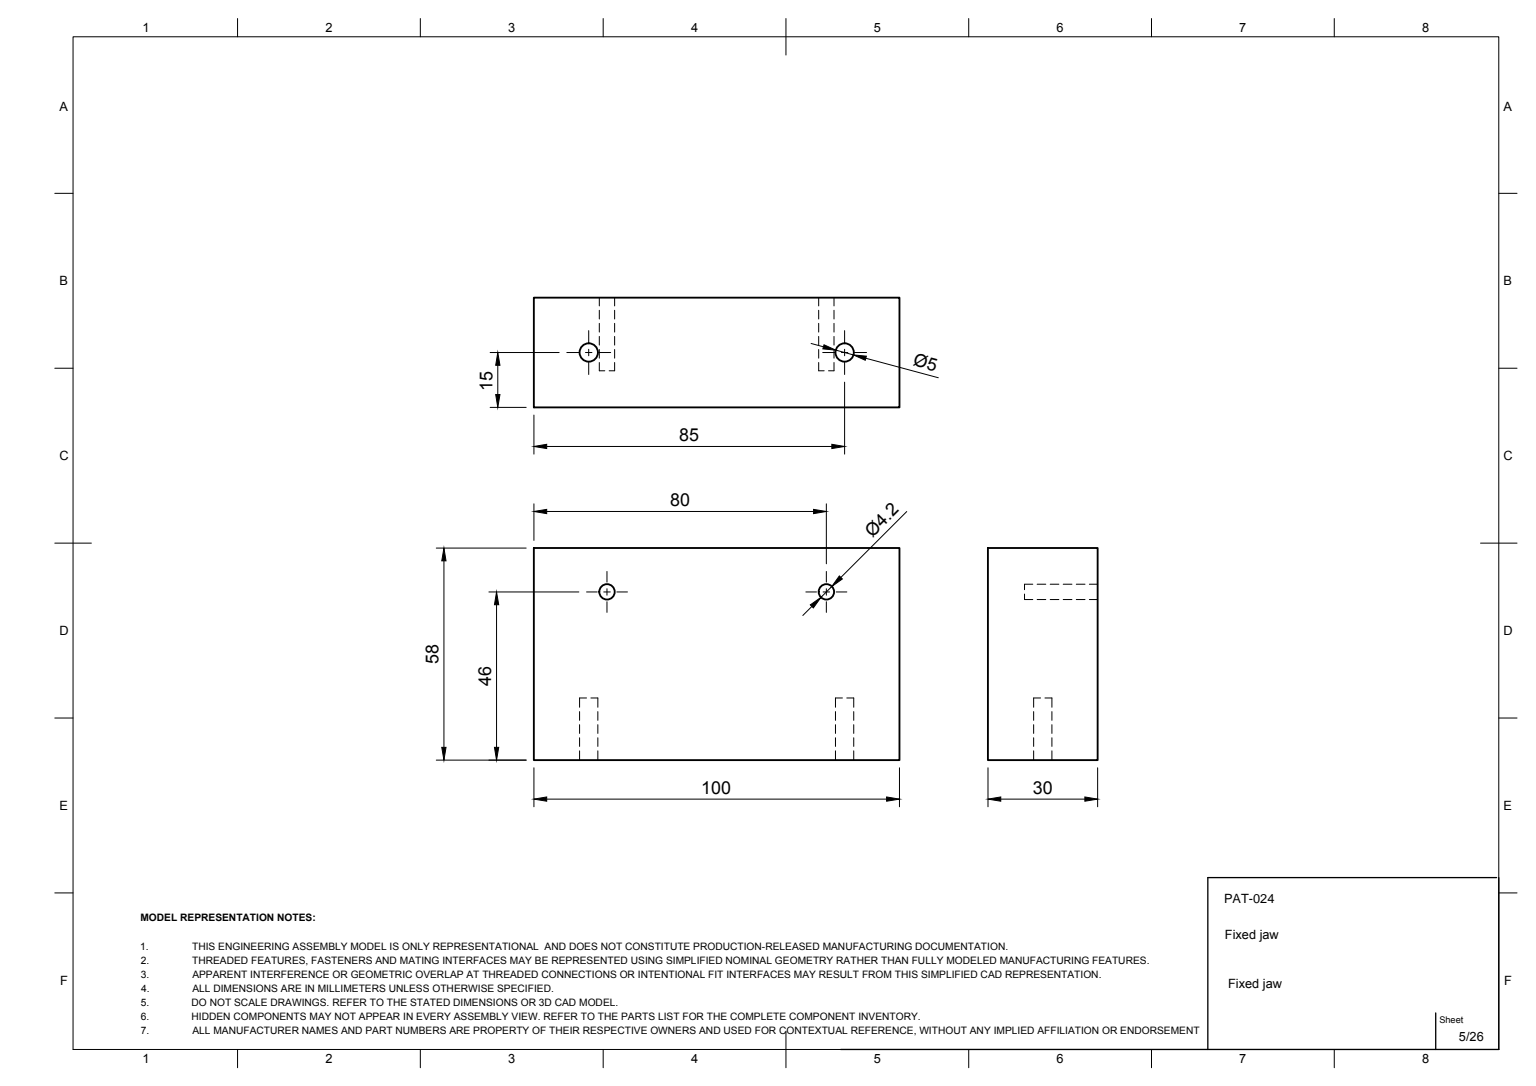
ISO-10303-21;
HEADER;
/* Generated by software containing ST-Developer
 * from STEP Tools, Inc. (www.steptools.com) 
 */

FILE_DESCRIPTION(
/* description */ ('Compact handwheel screw vise'),
/* implementation_level */ '2;1');

FILE_NAME(
/* name */ 'Fixed jaw.step',
/* time_stamp */ '2026-10-29T16:08:22-07:00',
/* author */ (''),
/* organization */ (''),
/* preprocessor_version */ 'ST-DEVELOPER v20.2',
/* originating_system */ 'Autodesk Translation Framework v15.17.0.0',
/* authorisation */ '');

FILE_SCHEMA (('AUTOMOTIVE_DESIGN { 1 0 10303 214 3 1 1 }'));
ENDSEC;

DATA;
#10=MECHANICAL_DESIGN_GEOMETRIC_PRESENTATION_REPRESENTATION('',(#646),#25074);
#590=SHAPE_REPRESENTATION_RELATIONSHIP('SRR','None',#25198,#618);
#618=ADVANCED_BREP_SHAPE_REPRESENTATION('',(#682),#25045);
#646=STYLED_ITEM('',(#25425),#682);
#682=MANIFOLD_SOLID_BREP('Body1',#8054);
#729=FACE_BOUND('',#1534,.T.);
#730=FACE_BOUND('',#1535,.T.);
#731=FACE_BOUND('',#1540,.T.);
#732=FACE_BOUND('',#1541,.T.);
#837=PLANE('',#8454);
#838=PLANE('',#8458);
#839=PLANE('',#8462);
#840=PLANE('',#8466);
#841=PLANE('',#8467);
#842=PLANE('',#8468);
#843=PLANE('',#8469);
#844=PLANE('',#8470);
#845=PLANE('',#8471);
#846=PLANE('',#8472);
#1037=FACE_OUTER_BOUND('',#1524,.T.);
#1038=FACE_OUTER_BOUND('',#1525,.T.);
#1039=FACE_OUTER_BOUND('',#1526,.T.);
#1040=FACE_OUTER_BOUND('',#1527,.T.);
#1041=FACE_OUTER_BOUND('',#1528,.T.);
#1042=FACE_OUTER_BOUND('',#1529,.T.);
#1043=FACE_OUTER_BOUND('',#1530,.T.);
#1044=FACE_OUTER_BOUND('',#1531,.T.);
#1045=FACE_OUTER_BOUND('',#1532,.T.);
#1046=FACE_OUTER_BOUND('',#1533,.T.);
#1047=FACE_OUTER_BOUND('',#1536,.T.);
#1048=FACE_OUTER_BOUND('',#1537,.T.);
#1049=FACE_OUTER_BOUND('',#1538,.T.);
#1050=FACE_OUTER_BOUND('',#1539,.T.);
#1524=EDGE_LOOP('',(#5267,#5268,#5269,#5270));
#1525=EDGE_LOOP('',(#5271));
#1526=EDGE_LOOP('',(#5272,#5273,#5274,#5275));
#1527=EDGE_LOOP('',(#5276));
#1528=EDGE_LOOP('',(#5277,#5278,#5279,#5280));
#1529=EDGE_LOOP('',(#5281));
#1530=EDGE_LOOP('',(#5282,#5283,#5284,#5285));
#1531=EDGE_LOOP('',(#5286));
#1532=EDGE_LOOP('',(#5287,#5288,#5289,#5290));
#1533=EDGE_LOOP('',(#5291,#5292,#5293,#5294));
#1534=EDGE_LOOP('',(#5295));
#1535=EDGE_LOOP('',(#5296));
#1536=EDGE_LOOP('',(#5297,#5298,#5299,#5300));
#1537=EDGE_LOOP('',(#5301,#5302,#5303,#5304));
#1538=EDGE_LOOP('',(#5305,#5306,#5307,#5308));
#1539=EDGE_LOOP('',(#5309,#5310,#5311,#5312));
#1540=EDGE_LOOP('',(#5313));
#1541=EDGE_LOOP('',(#5314));
#2096=LINE('',#11442,#2604);
#2097=LINE('',#11449,#2605);
#2098=LINE('',#11456,#2606);
#2099=LINE('',#11463,#2607);
#2100=LINE('',#11469,#2608);
#2101=LINE('',#11471,#2609);
#2102=LINE('',#11473,#2610);
#2103=LINE('',#11474,#2611);
#2104=LINE('',#11477,#2612);
#2105=LINE('',#11479,#2613);
#2106=LINE('',#11480,#2614);
#2107=LINE('',#11483,#2615);
#2108=LINE('',#11485,#2616);
#2109=LINE('',#11486,#2617);
#2110=LINE('',#11488,#2618);
#2111=LINE('',#11489,#2619);
#2604=VECTOR('',#9342,0.21);
#2605=VECTOR('',#9351,0.21);
#2606=VECTOR('',#9360,0.25);
#2607=VECTOR('',#9369,0.25);
#2608=VECTOR('',#9376,1.);
#2609=VECTOR('',#9377,1.);
#2610=VECTOR('',#9378,1.);
#2611=VECTOR('',#9379,1.);
#2612=VECTOR('',#9382,1.);
#2613=VECTOR('',#9383,1.);
#2614=VECTOR('',#9384,1.);
#2615=VECTOR('',#9387,1.);
#2616=VECTOR('',#9388,1.);
#2617=VECTOR('',#9389,1.);
#2618=VECTOR('',#9392,1.);
#2619=VECTOR('',#9393,1.);
#3098=CIRCLE('',#8452,0.21);
#3099=CIRCLE('',#8453,0.21);
#3100=CIRCLE('',#8456,0.21);
#3101=CIRCLE('',#8457,0.21);
#3102=CIRCLE('',#8460,0.25);
#3103=CIRCLE('',#8461,0.25);
#3104=CIRCLE('',#8464,0.25);
#3105=CIRCLE('',#8465,0.25);
#3369=VERTEX_POINT('',#11439);
#3370=VERTEX_POINT('',#11441);
#3371=VERTEX_POINT('',#11446);
#3372=VERTEX_POINT('',#11448);
#3373=VERTEX_POINT('',#11453);
#3374=VERTEX_POINT('',#11455);
#3375=VERTEX_POINT('',#11460);
#3376=VERTEX_POINT('',#11462);
#3377=VERTEX_POINT('',#11467);
#3378=VERTEX_POINT('',#11468);
#3379=VERTEX_POINT('',#11470);
#3380=VERTEX_POINT('',#11472);
#3381=VERTEX_POINT('',#11476);
#3382=VERTEX_POINT('',#11478);
#3383=VERTEX_POINT('',#11482);
#3384=VERTEX_POINT('',#11484);
#4120=EDGE_CURVE('',#3369,#3369,#3098,.T.);
#4121=EDGE_CURVE('',#3369,#3370,#2096,.T.);
#4122=EDGE_CURVE('',#3370,#3370,#3099,.T.);
#4123=EDGE_CURVE('',#3371,#3371,#3100,.T.);
#4124=EDGE_CURVE('',#3371,#3372,#2097,.T.);
#4125=EDGE_CURVE('',#3372,#3372,#3101,.T.);
#4126=EDGE_CURVE('',#3373,#3373,#3102,.T.);
#4127=EDGE_CURVE('',#3373,#3374,#2098,.T.);
#4128=EDGE_CURVE('',#3374,#3374,#3103,.T.);
#4129=EDGE_CURVE('',#3375,#3375,#3104,.T.);
#4130=EDGE_CURVE('',#3375,#3376,#2099,.T.);
#4131=EDGE_CURVE('',#3376,#3376,#3105,.T.);
#4132=EDGE_CURVE('',#3377,#3378,#2100,.T.);
#4133=EDGE_CURVE('',#3378,#3379,#2101,.T.);
#4134=EDGE_CURVE('',#3380,#3379,#2102,.T.);
#4135=EDGE_CURVE('',#3377,#3380,#2103,.T.);
#4136=EDGE_CURVE('',#3381,#3377,#2104,.T.);
#4137=EDGE_CURVE('',#3382,#3380,#2105,.T.);
#4138=EDGE_CURVE('',#3381,#3382,#2106,.T.);
#4139=EDGE_CURVE('',#3383,#3381,#2107,.T.);
#4140=EDGE_CURVE('',#3384,#3382,#2108,.T.);
#4141=EDGE_CURVE('',#3383,#3384,#2109,.T.);
#4142=EDGE_CURVE('',#3378,#3383,#2110,.T.);
#4143=EDGE_CURVE('',#3379,#3384,#2111,.T.);
#5267=ORIENTED_EDGE('',*,*,#4120,.F.);
#5268=ORIENTED_EDGE('',*,*,#4121,.T.);
#5269=ORIENTED_EDGE('',*,*,#4122,.F.);
#5270=ORIENTED_EDGE('',*,*,#4121,.F.);
#5271=ORIENTED_EDGE('',*,*,#4120,.T.);
#5272=ORIENTED_EDGE('',*,*,#4123,.F.);
#5273=ORIENTED_EDGE('',*,*,#4124,.T.);
#5274=ORIENTED_EDGE('',*,*,#4125,.F.);
#5275=ORIENTED_EDGE('',*,*,#4124,.F.);
#5276=ORIENTED_EDGE('',*,*,#4123,.T.);
#5277=ORIENTED_EDGE('',*,*,#4126,.F.);
#5278=ORIENTED_EDGE('',*,*,#4127,.T.);
#5279=ORIENTED_EDGE('',*,*,#4128,.T.);
#5280=ORIENTED_EDGE('',*,*,#4127,.F.);
#5281=ORIENTED_EDGE('',*,*,#4128,.F.);
#5282=ORIENTED_EDGE('',*,*,#4129,.F.);
#5283=ORIENTED_EDGE('',*,*,#4130,.T.);
#5284=ORIENTED_EDGE('',*,*,#4131,.T.);
#5285=ORIENTED_EDGE('',*,*,#4130,.F.);
#5286=ORIENTED_EDGE('',*,*,#4131,.F.);
#5287=ORIENTED_EDGE('',*,*,#4132,.T.);
#5288=ORIENTED_EDGE('',*,*,#4133,.T.);
#5289=ORIENTED_EDGE('',*,*,#4134,.F.);
#5290=ORIENTED_EDGE('',*,*,#4135,.F.);
#5291=ORIENTED_EDGE('',*,*,#4136,.T.);
#5292=ORIENTED_EDGE('',*,*,#4135,.T.);
#5293=ORIENTED_EDGE('',*,*,#4137,.F.);
#5294=ORIENTED_EDGE('',*,*,#4138,.F.);
#5295=ORIENTED_EDGE('',*,*,#4122,.T.);
#5296=ORIENTED_EDGE('',*,*,#4125,.T.);
#5297=ORIENTED_EDGE('',*,*,#4139,.T.);
#5298=ORIENTED_EDGE('',*,*,#4138,.T.);
#5299=ORIENTED_EDGE('',*,*,#4140,.F.);
#5300=ORIENTED_EDGE('',*,*,#4141,.F.);
#5301=ORIENTED_EDGE('',*,*,#4142,.T.);
#5302=ORIENTED_EDGE('',*,*,#4141,.T.);
#5303=ORIENTED_EDGE('',*,*,#4143,.F.);
#5304=ORIENTED_EDGE('',*,*,#4133,.F.);
#5305=ORIENTED_EDGE('',*,*,#4143,.T.);
#5306=ORIENTED_EDGE('',*,*,#4140,.T.);
#5307=ORIENTED_EDGE('',*,*,#4137,.T.);
#5308=ORIENTED_EDGE('',*,*,#4134,.T.);
#5309=ORIENTED_EDGE('',*,*,#4142,.F.);
#5310=ORIENTED_EDGE('',*,*,#4132,.F.);
#5311=ORIENTED_EDGE('',*,*,#4136,.F.);
#5312=ORIENTED_EDGE('',*,*,#4139,.F.);
#5313=ORIENTED_EDGE('',*,*,#4126,.T.);
#5314=ORIENTED_EDGE('',*,*,#4129,.T.);
#7355=CYLINDRICAL_SURFACE('',#8451,0.21);
#7356=CYLINDRICAL_SURFACE('',#8455,0.21);
#7357=CYLINDRICAL_SURFACE('',#8459,0.25);
#7358=CYLINDRICAL_SURFACE('',#8463,0.25);
#7607=ADVANCED_FACE('',(#1037),#7355,.F.);
#7608=ADVANCED_FACE('',(#1038),#837,.T.);
#7609=ADVANCED_FACE('',(#1039),#7356,.F.);
#7610=ADVANCED_FACE('',(#1040),#838,.T.);
#7611=ADVANCED_FACE('',(#1041),#7357,.F.);
#7612=ADVANCED_FACE('',(#1042),#839,.F.);
#7613=ADVANCED_FACE('',(#1043),#7358,.F.);
#7614=ADVANCED_FACE('',(#1044),#840,.F.);
#7615=ADVANCED_FACE('',(#1045),#841,.T.);
#7616=ADVANCED_FACE('',(#1046,#729,#730),#842,.T.);
#7617=ADVANCED_FACE('',(#1047),#843,.T.);
#7618=ADVANCED_FACE('',(#1048),#844,.T.);
#7619=ADVANCED_FACE('',(#1049),#845,.T.);
#7620=ADVANCED_FACE('',(#1050,#731,#732),#846,.F.);
#8054=CLOSED_SHELL('',(#7607,#7608,#7609,#7610,#7611,#7612,#7613,#7614,
#7615,#7616,#7617,#7618,#7619,#7620));
#8450=AXIS2_PLACEMENT_3D('',#11437,#9336,#9337);
#8451=AXIS2_PLACEMENT_3D('',#11438,#9338,#9339);
#8452=AXIS2_PLACEMENT_3D('',#11440,#9340,#9341);
#8453=AXIS2_PLACEMENT_3D('',#11443,#9343,#9344);
#8454=AXIS2_PLACEMENT_3D('',#11444,#9345,#9346);
#8455=AXIS2_PLACEMENT_3D('',#11445,#9347,#9348);
#8456=AXIS2_PLACEMENT_3D('',#11447,#9349,#9350);
#8457=AXIS2_PLACEMENT_3D('',#11450,#9352,#9353);
#8458=AXIS2_PLACEMENT_3D('',#11451,#9354,#9355);
#8459=AXIS2_PLACEMENT_3D('',#11452,#9356,#9357);
#8460=AXIS2_PLACEMENT_3D('',#11454,#9358,#9359);
#8461=AXIS2_PLACEMENT_3D('',#11457,#9361,#9362);
#8462=AXIS2_PLACEMENT_3D('',#11458,#9363,#9364);
#8463=AXIS2_PLACEMENT_3D('',#11459,#9365,#9366);
#8464=AXIS2_PLACEMENT_3D('',#11461,#9367,#9368);
#8465=AXIS2_PLACEMENT_3D('',#11464,#9370,#9371);
#8466=AXIS2_PLACEMENT_3D('',#11465,#9372,#9373);
#8467=AXIS2_PLACEMENT_3D('',#11466,#9374,#9375);
#8468=AXIS2_PLACEMENT_3D('',#11475,#9380,#9381);
#8469=AXIS2_PLACEMENT_3D('',#11481,#9385,#9386);
#8470=AXIS2_PLACEMENT_3D('',#11487,#9390,#9391);
#8471=AXIS2_PLACEMENT_3D('',#11490,#9394,#9395);
#8472=AXIS2_PLACEMENT_3D('',#11491,#9396,#9397);
#9336=DIRECTION('axis',(0.,0.,1.));
#9337=DIRECTION('refdir',(1.,0.,0.));
#9338=DIRECTION('center_axis',(1.,0.,0.));
#9339=DIRECTION('ref_axis',(0.,0.,-1.));
#9340=DIRECTION('center_axis',(1.,0.,0.));
#9341=DIRECTION('ref_axis',(0.,0.,-1.));
#9342=DIRECTION('',(1.,0.,0.));
#9343=DIRECTION('center_axis',(-1.,0.,0.));
#9344=DIRECTION('ref_axis',(0.,0.,-1.));
#9345=DIRECTION('center_axis',(1.,0.,0.));
#9346=DIRECTION('ref_axis',(0.,0.,-1.));
#9347=DIRECTION('center_axis',(1.,0.,0.));
#9348=DIRECTION('ref_axis',(0.,0.,-1.));
#9349=DIRECTION('center_axis',(1.,0.,0.));
#9350=DIRECTION('ref_axis',(0.,0.,-1.));
#9351=DIRECTION('',(1.,0.,0.));
#9352=DIRECTION('center_axis',(-1.,0.,0.));
#9353=DIRECTION('ref_axis',(0.,0.,-1.));
#9354=DIRECTION('center_axis',(1.,0.,0.));
#9355=DIRECTION('ref_axis',(0.,0.,-1.));
#9356=DIRECTION('center_axis',(0.,0.,1.));
#9357=DIRECTION('ref_axis',(1.,0.,0.));
#9358=DIRECTION('center_axis',(0.,0.,1.));
#9359=DIRECTION('ref_axis',(1.,0.,0.));
#9360=DIRECTION('',(0.,0.,1.));
#9361=DIRECTION('center_axis',(0.,0.,1.));
#9362=DIRECTION('ref_axis',(1.,0.,0.));
#9363=DIRECTION('center_axis',(0.,0.,1.));
#9364=DIRECTION('ref_axis',(1.,0.,0.));
#9365=DIRECTION('center_axis',(0.,0.,1.));
#9366=DIRECTION('ref_axis',(1.,0.,0.));
#9367=DIRECTION('center_axis',(0.,0.,1.));
#9368=DIRECTION('ref_axis',(1.,0.,0.));
#9369=DIRECTION('',(0.,0.,1.));
#9370=DIRECTION('center_axis',(0.,0.,1.));
#9371=DIRECTION('ref_axis',(1.,0.,0.));
#9372=DIRECTION('center_axis',(0.,0.,1.));
#9373=DIRECTION('ref_axis',(1.,0.,0.));
#9374=DIRECTION('center_axis',(0.,1.,0.));
#9375=DIRECTION('ref_axis',(-1.,0.,0.));
#9376=DIRECTION('',(-1.,0.,0.));
#9377=DIRECTION('',(0.,0.,1.));
#9378=DIRECTION('',(-1.,0.,0.));
#9379=DIRECTION('',(0.,0.,1.));
#9380=DIRECTION('center_axis',(1.,0.,0.));
#9381=DIRECTION('ref_axis',(0.,1.,0.));
#9382=DIRECTION('',(0.,1.,0.));
#9383=DIRECTION('',(0.,1.,0.));
#9384=DIRECTION('',(0.,0.,1.));
#9385=DIRECTION('center_axis',(0.,-1.,0.));
#9386=DIRECTION('ref_axis',(1.,0.,0.));
#9387=DIRECTION('',(1.,0.,0.));
#9388=DIRECTION('',(1.,0.,0.));
#9389=DIRECTION('',(0.,0.,1.));
#9390=DIRECTION('center_axis',(-1.,0.,0.));
#9391=DIRECTION('ref_axis',(0.,-1.,0.));
#9392=DIRECTION('',(0.,-1.,0.));
#9393=DIRECTION('',(0.,-1.,0.));
#9394=DIRECTION('center_axis',(0.,0.,1.));
#9395=DIRECTION('ref_axis',(1.,0.,0.));
#9396=DIRECTION('center_axis',(0.,0.,1.));
#9397=DIRECTION('ref_axis',(1.,0.,0.));
#11437=CARTESIAN_POINT('',(0.,0.,0.));
#11438=CARTESIAN_POINT('Origin',(1.,-3.,5.8));
#11439=CARTESIAN_POINT('',(1.,-3.,6.01));
#11440=CARTESIAN_POINT('Origin',(1.,-3.,5.8));
#11441=CARTESIAN_POINT('',(3.,-3.,6.01));
#11442=CARTESIAN_POINT('',(1.,-3.,6.01));
#11443=CARTESIAN_POINT('Origin',(3.,-3.,5.8));
#11444=CARTESIAN_POINT('Origin',(1.,-3.,5.8));
#11445=CARTESIAN_POINT('Origin',(1.,3.,5.8));
#11446=CARTESIAN_POINT('',(1.,3.,6.01));
#11447=CARTESIAN_POINT('Origin',(1.,3.,5.8));
#11448=CARTESIAN_POINT('',(3.,3.,6.01));
#11449=CARTESIAN_POINT('',(1.,3.,6.01));
#11450=CARTESIAN_POINT('Origin',(3.,3.,5.8));
#11451=CARTESIAN_POINT('Origin',(1.,3.,5.8));
#11452=CARTESIAN_POINT('Origin',(1.5,-3.5,1.1));
#11453=CARTESIAN_POINT('',(1.25,-3.5,1.2));
#11454=CARTESIAN_POINT('Origin',(1.5,-3.5,1.2));
#11455=CARTESIAN_POINT('',(1.25,-3.5,2.9));
#11456=CARTESIAN_POINT('',(1.25,-3.5,1.1));
#11457=CARTESIAN_POINT('Origin',(1.5,-3.5,2.9));
#11458=CARTESIAN_POINT('Origin',(1.5,-3.5,2.9));
#11459=CARTESIAN_POINT('Origin',(1.5,3.5,1.1));
#11460=CARTESIAN_POINT('',(1.25,3.5,1.2));
#11461=CARTESIAN_POINT('Origin',(1.5,3.5,1.2));
#11462=CARTESIAN_POINT('',(1.25,3.5,2.9));
#11463=CARTESIAN_POINT('',(1.25,3.5,1.1));
#11464=CARTESIAN_POINT('Origin',(1.5,3.5,2.9));
#11465=CARTESIAN_POINT('Origin',(1.5,3.5,2.9));
#11466=CARTESIAN_POINT('Origin',(3.,5.,1.2));
#11467=CARTESIAN_POINT('',(3.,5.,1.2));
#11468=CARTESIAN_POINT('',(0.,5.,1.2));
#11469=CARTESIAN_POINT('',(3.,5.,1.2));
#11470=CARTESIAN_POINT('',(0.,5.,7.));
#11471=CARTESIAN_POINT('',(0.,5.,1.2));
#11472=CARTESIAN_POINT('',(3.,5.,7.));
#11473=CARTESIAN_POINT('',(3.,5.,7.));
#11474=CARTESIAN_POINT('',(3.,5.,1.2));
#11475=CARTESIAN_POINT('Origin',(3.,-5.,1.2));
#11476=CARTESIAN_POINT('',(3.,-5.,1.2));
#11477=CARTESIAN_POINT('',(3.,-5.,1.2));
#11478=CARTESIAN_POINT('',(3.,-5.,7.));
#11479=CARTESIAN_POINT('',(3.,-5.,7.));
#11480=CARTESIAN_POINT('',(3.,-5.,1.2));
#11481=CARTESIAN_POINT('Origin',(0.,-5.,1.2));
#11482=CARTESIAN_POINT('',(0.,-5.,1.2));
#11483=CARTESIAN_POINT('',(0.,-5.,1.2));
#11484=CARTESIAN_POINT('',(0.,-5.,7.));
#11485=CARTESIAN_POINT('',(0.,-5.,7.));
#11486=CARTESIAN_POINT('',(0.,-5.,1.2));
#11487=CARTESIAN_POINT('Origin',(0.,5.,1.2));
#11488=CARTESIAN_POINT('',(0.,5.,1.2));
#11489=CARTESIAN_POINT('',(0.,5.,7.));
#11490=CARTESIAN_POINT('Origin',(1.5,0.,7.));
#11491=CARTESIAN_POINT('Origin',(1.5,0.,1.2));
#25011=UNCERTAINTY_MEASURE_WITH_UNIT(LENGTH_MEASURE(0.001),#25075,
'DISTANCE_ACCURACY_VALUE',
'Maximum model space distance between geometric entities at asserted c
onnectivities');
#25040=UNCERTAINTY_MEASURE_WITH_UNIT(LENGTH_MEASURE(0.001),#25075,
'DISTANCE_ACCURACY_VALUE',
'Maximum model space distance between geometric entities at asserted c
onnectivities');
#25045=(
GEOMETRIC_REPRESENTATION_CONTEXT(3)
GLOBAL_UNCERTAINTY_ASSIGNED_CONTEXT((#25011))
GLOBAL_UNIT_ASSIGNED_CONTEXT((#25075,#25077,#25078))
REPRESENTATION_CONTEXT('','3D')
);
#25074=(
GEOMETRIC_REPRESENTATION_CONTEXT(3)
GLOBAL_UNCERTAINTY_ASSIGNED_CONTEXT((#25040))
GLOBAL_UNIT_ASSIGNED_CONTEXT((#25075,#25077,#25078))
REPRESENTATION_CONTEXT('','3D')
);
#25075=(
LENGTH_UNIT()
NAMED_UNIT(*)
SI_UNIT(.CENTI.,.METRE.)
);
#25077=(
NAMED_UNIT(*)
PLANE_ANGLE_UNIT()
SI_UNIT($,.RADIAN.)
);
#25078=(
NAMED_UNIT(*)
SI_UNIT($,.STERADIAN.)
SOLID_ANGLE_UNIT()
);
#25083=SHAPE_DEFINITION_REPRESENTATION(#25116,#25198);
#25116=PRODUCT_DEFINITION_SHAPE('',$,#25232);
#25198=SHAPE_REPRESENTATION('',(#8450),#25045);
#25227=PRODUCT_DEFINITION_CONTEXT('part definition',#25328,'design');
#25232=PRODUCT_DEFINITION('Fixed jaw','Fixed jaw',#25265,#25227);
#25265=PRODUCT_DEFINITION_FORMATION('',$,#25334);
#25328=APPLICATION_CONTEXT(
'Core Data for Automotive Mechanical Design Process');
#25329=PRODUCT_CONTEXT('part definition',#25328,'mechanical');
#25334=PRODUCT('Fixed jaw','Fixed jaw','Fixed jaw',(#25329));
#25419=COLOUR_RGB('Light Blue',0.38,0.62,0.78);
#25420=FILL_AREA_STYLE_COLOUR('',#25419);
#25421=FILL_AREA_STYLE('',(#25420));
#25422=SURFACE_STYLE_FILL_AREA(#25421);
#25423=SURFACE_SIDE_STYLE('',(#25422));
#25424=SURFACE_STYLE_USAGE(.BOTH.,#25423);
#25425=PRESENTATION_STYLE_ASSIGNMENT((#25424));
ENDSEC;
END-ISO-10303-21;
